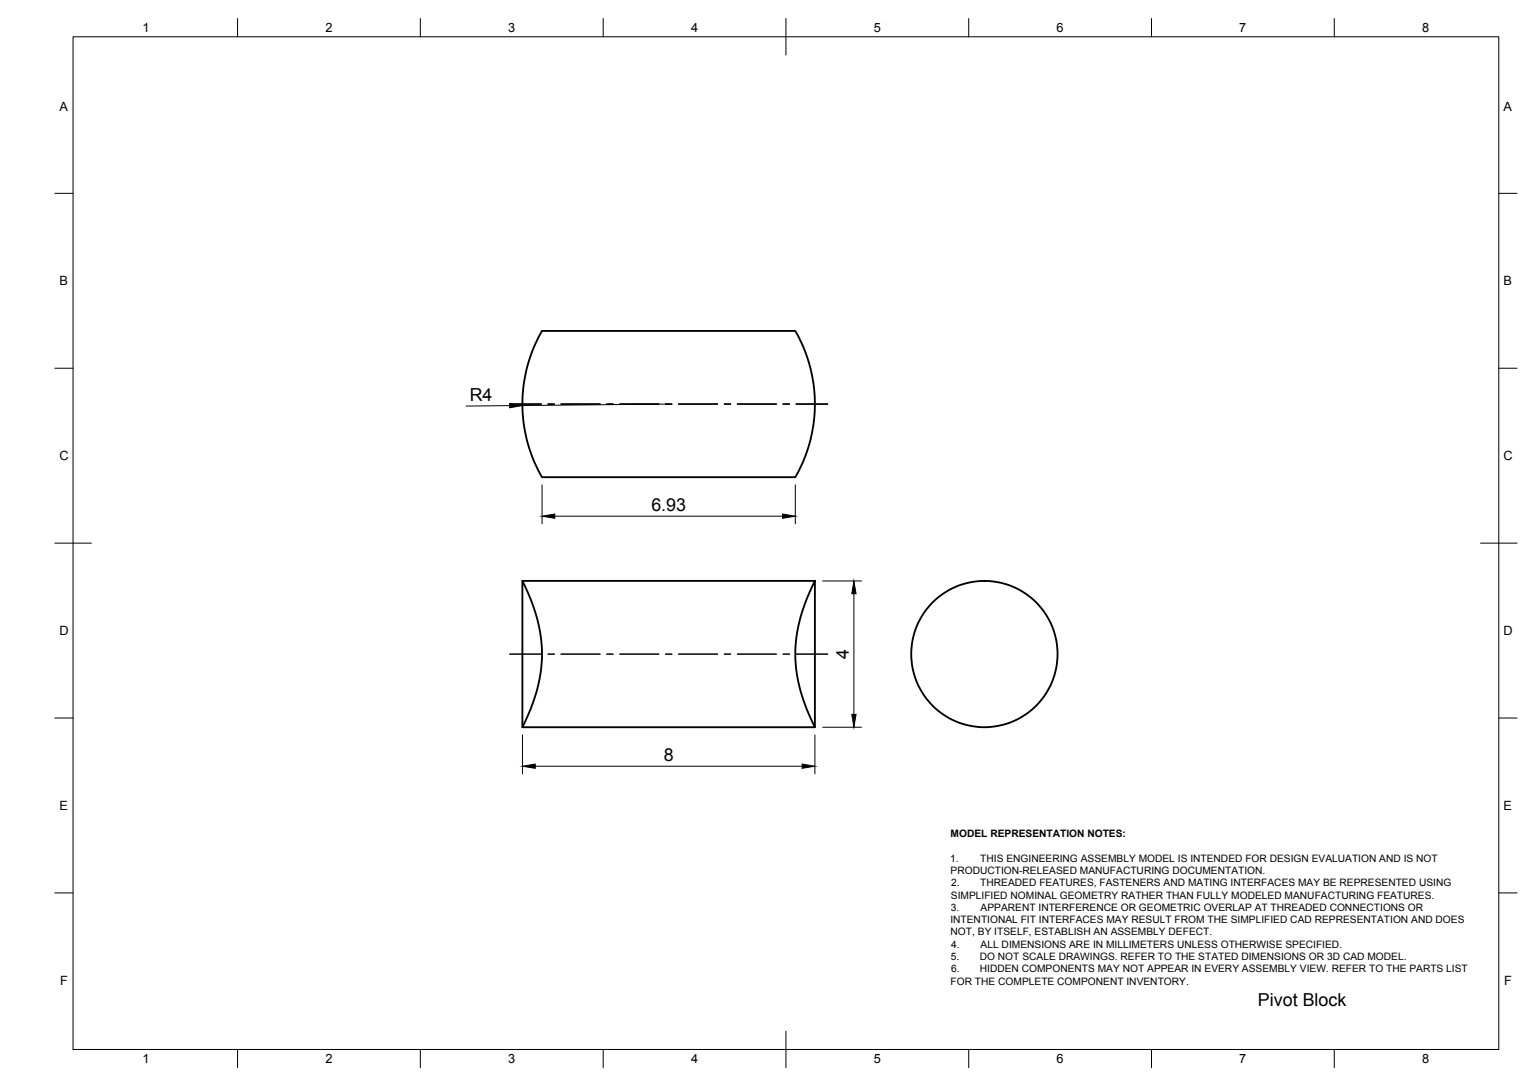
ISO-10303-21;
HEADER;
/* Generated by software containing ST-Developer
 * from STEP Tools, Inc. (www.steptools.com) 
 */

FILE_DESCRIPTION(
/* description */ ('STEP AP214'),
/* implementation_level */ '2;1');

FILE_NAME(
/* name */ 'Pivot Block.step',
/* time_stamp */ '2026-10-06T11:11:25-07:00',
/* author */ (''),
/* organization */ (''),
/* preprocessor_version */ 'ST-DEVELOPER v20.2',
/* originating_system */ 'Autodesk Translation Framework v15.15.0.0',
/* authorisation */ '');

FILE_SCHEMA (('AUTOMOTIVE_DESIGN { 1 0 10303 214 3 1 1 }'));
ENDSEC;

DATA;
#10=MECHANICAL_DESIGN_GEOMETRIC_PRESENTATION_REPRESENTATION('',(#703),#47717);
#450=B_SPLINE_CURVE_WITH_KNOTS('',3,(#44279,#44280,#44281,#44282,#44283,
#44284,#44285,#44286,#44287,#44288,#44289,#44290,#44291,#44292,#44293,#44294,
#44295,#44296,#44297,#44298,#44299,#44300,#44301,#44302,#44303,#44304,#44305),
 .UNSPECIFIED.,.F.,.F.,(4,2,2,2,3,2,2,2,2,2,2,2,4),(0.922537325049047,0.999310505714261,
1.07608368637947,1.15306672655577,1.23004976673206,1.30703280690836,1.38401584708465,
1.46078902774986,1.53756220841508,1.61433538908029,1.69110856974551,1.7680916099218,
1.84507465009809),.UNSPECIFIED.);
#451=B_SPLINE_CURVE_WITH_KNOTS('',3,(#44306,#44307,#44308,#44309,#44310,
#44311,#44312,#44313,#44314,#44315),.UNSPECIFIED.,.F.,.F.,(4,2,2,2,4),(1.84507465009809,
1.92205769027439,1.99904073045068,2.0758139111159,2.15258709178111),
 .UNSPECIFIED.);
#452=B_SPLINE_CURVE_WITH_KNOTS('',3,(#44318,#44319,#44320,#44321,#44322,
#44323,#44324,#44325,#44326,#44327,#44328,#44329,#44330,#44331,#44332,#44333,
#44334,#44335,#44336,#44337,#44338,#44339,#44340,#44341,#44342,#44343,#44344,
#44345,#44346,#44347,#44348,#44349,#44350,#44351),.UNSPECIFIED.,.T.,.F.,
(4,2,2,2,2,2,2,2,2,2,2,2,2,2,2,2,4),(-1.23004976673206,-1.15306672655577,
-1.07608368637947,-0.999310505714261,-0.922537325049047,-0.845764144383833,
-0.76899096371862,-0.692007923542325,-0.615024883366031,-0.538041843189737,
-0.461058803013443,-0.384285622348229,-0.307512441683016,-0.230739261017802,
-0.153966080352588,-0.0769830401762941,0.),.UNSPECIFIED.);
#679=SHAPE_REPRESENTATION_RELATIONSHIP('SRR','None',#47766,#691);
#691=ADVANCED_BREP_SHAPE_REPRESENTATION('',(#715),#47710);
#703=STYLED_ITEM('',(#47830),#715);
#715=MANIFOLD_SOLID_BREP('Body1',#8930);
#1145=LINE('',#44352,#1632);
#1632=VECTOR('',#11106,2.);
#1995=CYLINDRICAL_SURFACE('',#9512,4.);
#1996=CYLINDRICAL_SURFACE('',#9513,2.);
#1997=CYLINDRICAL_SURFACE('',#9514,4.);
#2360=FACE_OUTER_BOUND('',#2881,.T.);
#2361=FACE_OUTER_BOUND('',#2882,.T.);
#2362=FACE_OUTER_BOUND('',#2883,.T.);
#2881=EDGE_LOOP('',(#7339,#7340));
#2882=EDGE_LOOP('',(#7341,#7342,#7343,#7344,#7345));
#2883=EDGE_LOOP('',(#7346));
#4056=VERTEX_POINT('',#44277);
#4057=VERTEX_POINT('',#44278);
#4058=VERTEX_POINT('',#44317);
#5195=EDGE_CURVE('',#4056,#4057,#450,.T.);
#5196=EDGE_CURVE('',#4057,#4056,#451,.T.);
#5197=EDGE_CURVE('',#4058,#4058,#452,.T.);
#5198=EDGE_CURVE('',#4058,#4057,#1145,.T.);
#7339=ORIENTED_EDGE('',*,*,#5195,.T.);
#7340=ORIENTED_EDGE('',*,*,#5196,.T.);
#7341=ORIENTED_EDGE('',*,*,#5197,.F.);
#7342=ORIENTED_EDGE('',*,*,#5198,.T.);
#7343=ORIENTED_EDGE('',*,*,#5195,.F.);
#7344=ORIENTED_EDGE('',*,*,#5196,.F.);
#7345=ORIENTED_EDGE('',*,*,#5198,.F.);
#7346=ORIENTED_EDGE('',*,*,#5197,.T.);
#8710=ADVANCED_FACE('',(#2360),#1995,.T.);
#8711=ADVANCED_FACE('',(#2361),#1996,.T.);
#8712=ADVANCED_FACE('',(#2362),#1997,.T.);
#8930=CLOSED_SHELL('',(#8710,#8711,#8712));
#9511=AXIS2_PLACEMENT_3D('',#44275,#11100,#11101);
#9512=AXIS2_PLACEMENT_3D('',#44276,#11102,#11103);
#9513=AXIS2_PLACEMENT_3D('',#44316,#11104,#11105);
#9514=AXIS2_PLACEMENT_3D('',#44353,#11107,#11108);
#11100=DIRECTION('axis',(0.,0.,1.));
#11101=DIRECTION('refdir',(1.,0.,0.));
#11102=DIRECTION('center_axis',(0.106006004448152,0.994365489657067,0.));
#11103=DIRECTION('ref_axis',(0.,0.,1.));
#11104=DIRECTION('center_axis',(0.,0.,-1.));
#11105=DIRECTION('ref_axis',(-0.994365489657067,0.106006004448153,0.));
#11106=DIRECTION('',(0.,0.,1.));
#11107=DIRECTION('center_axis',(0.106006004448152,0.994365489657067,0.));
#11108=DIRECTION('ref_axis',(1.21774651409112E-16,-1.29819914037829E-17,
-1.));
#44275=CARTESIAN_POINT('',(0.,0.,0.));
#44276=CARTESIAN_POINT('Origin',(-53.8258982150057,-64.4396735761727,175.985485069079));
#44277=CARTESIAN_POINT('',(-53.4018741972131,-60.4622116175444,179.985485069079));
#44278=CARTESIAN_POINT('',(-51.6251552267953,-62.6629546057548,179.449586684217));
#44279=CARTESIAN_POINT('Ctrl Pts',(-53.4018741972131,-60.4622116175444,
179.985485069079));
#44280=CARTESIAN_POINT('Ctrl Pts',(-53.6563428684955,-60.4350835571074,
179.985485069079));
#44281=CARTESIAN_POINT('Ctrl Pts',(-53.9303211793164,-60.458242890839,179.958669005781));
#44282=CARTESIAN_POINT('Ctrl Pts',(-54.4409372535361,-60.6105704641806,
179.862014751158));
#44283=CARTESIAN_POINT('Ctrl Pts',(-54.6778490486358,-60.7394791031505,
179.79321828922));
#44284=CARTESIAN_POINT('Ctrl Pts',(-55.0631092638411,-61.0505100306915,
179.660886004177));
#44285=CARTESIAN_POINT('Ctrl Pts',(-55.2387001635013,-61.2547981540133,
179.587877094001));
#44286=CARTESIAN_POINT('Ctrl Pts',(-55.4948940947938,-61.7211552694728,
179.481135940985));
#44287=CARTESIAN_POINT('Ctrl Pts',(-55.5754149704257,-61.9837663264949,
179.449586684217));
#44288=CARTESIAN_POINT('Ctrl Pts',(-55.6026171854236,-62.2389305879622,
179.449586684217));
#44289=CARTESIAN_POINT('Ctrl Pts',(-55.6298194004214,-62.4940948494295,
179.449586684217));
#44290=CARTESIAN_POINT('Ctrl Pts',(-55.6064711817378,-62.7677790458441,
179.481135940985));
#44291=CARTESIAN_POINT('Ctrl Pts',(-55.4543512989582,-63.2776651417851,
179.587877094001));
#44292=CARTESIAN_POINT('Ctrl Pts',(-55.3257742211671,-63.5143796036173,
179.660886004177));
#44293=CARTESIAN_POINT('Ctrl Pts',(-55.0147432936261,-63.8996398188226,
179.79321828922));
#44294=CARTESIAN_POINT('Ctrl Pts',(-54.8103321708864,-64.0755964292659,
179.862014751158));
#44295=CARTESIAN_POINT('Ctrl Pts',(-54.343305267868,-64.3321472755105,179.958669005781));
#44296=CARTESIAN_POINT('Ctrl Pts',(-54.080366886288,-64.4125455157357,179.985485069079));
#44297=CARTESIAN_POINT('Ctrl Pts',(-53.5714295437234,-64.4668016366096,
179.985485069079));
#44298=CARTESIAN_POINT('Ctrl Pts',(-53.2974512329025,-64.443642302878,179.958669005781));
#44299=CARTESIAN_POINT('Ctrl Pts',(-52.7868351586827,-64.2913147295365,
179.862014751158));
#44300=CARTESIAN_POINT('Ctrl Pts',(-52.549923363583,-64.1624060905666,179.79321828922));
#44301=CARTESIAN_POINT('Ctrl Pts',(-52.1646631483778,-63.8513751630256,
179.660886004177));
#44302=CARTESIAN_POINT('Ctrl Pts',(-51.9890722487176,-63.6470870397037,
179.587877094001));
#44303=CARTESIAN_POINT('Ctrl Pts',(-51.732878317425,-63.1807299242443,179.481135940985));
#44304=CARTESIAN_POINT('Ctrl Pts',(-51.6523574417932,-62.9181188672221,
179.449586684217));
#44305=CARTESIAN_POINT('Ctrl Pts',(-51.6251552267953,-62.6629546057548,
179.449586684217));
#44306=CARTESIAN_POINT('Ctrl Pts',(-51.6251552267953,-62.6629546057548,
179.449586684217));
#44307=CARTESIAN_POINT('Ctrl Pts',(-51.5979530117974,-62.4077903442875,
179.449586684217));
#44308=CARTESIAN_POINT('Ctrl Pts',(-51.6213012304811,-62.1341061478729,
179.481135940985));
#44309=CARTESIAN_POINT('Ctrl Pts',(-51.7734211132606,-61.6242200519319,
179.587877094001));
#44310=CARTESIAN_POINT('Ctrl Pts',(-51.9019981910518,-61.3875055900997,
179.660886004177));
#44311=CARTESIAN_POINT('Ctrl Pts',(-52.2130291185928,-61.0022453748944,
179.79321828922));
#44312=CARTESIAN_POINT('Ctrl Pts',(-52.4174402413325,-60.8262887644511,
179.862014751158));
#44313=CARTESIAN_POINT('Ctrl Pts',(-52.8844671443509,-60.5697379182066,
179.958669005781));
#44314=CARTESIAN_POINT('Ctrl Pts',(-53.1474055259308,-60.4893396779814,
179.985485069079));
#44315=CARTESIAN_POINT('Ctrl Pts',(-53.4018741972131,-60.4622116175444,
179.985485069079));
#44316=CARTESIAN_POINT('Origin',(-53.6138862061094,-62.4509425968585,185.985485069079));
#44317=CARTESIAN_POINT('',(-51.6251552267953,-62.6629546057548,172.521383453942));
#44318=CARTESIAN_POINT('Ctrl Pts',(-55.6026171854236,-62.2389305879622,
172.521383453942));
#44319=CARTESIAN_POINT('Ctrl Pts',(-55.5754149704257,-61.9837663264949,
172.521383453942));
#44320=CARTESIAN_POINT('Ctrl Pts',(-55.4948940947938,-61.7211552694728,
172.489834197174));
#44321=CARTESIAN_POINT('Ctrl Pts',(-55.2387001635013,-61.2547981540133,
172.383093044158));
#44322=CARTESIAN_POINT('Ctrl Pts',(-55.0631092638411,-61.0505100306915,
172.310084133982));
#44323=CARTESIAN_POINT('Ctrl Pts',(-54.6778490486358,-60.7394791031505,
172.177751848938));
#44324=CARTESIAN_POINT('Ctrl Pts',(-54.4409372535361,-60.6105704641806,
172.108955387));
#44325=CARTESIAN_POINT('Ctrl Pts',(-53.9303211793164,-60.458242890839,172.012301132378));
#44326=CARTESIAN_POINT('Ctrl Pts',(-53.6563428684955,-60.4350835571074,
171.985485069079));
#44327=CARTESIAN_POINT('Ctrl Pts',(-53.1474055259308,-60.4893396779814,
171.985485069079));
#44328=CARTESIAN_POINT('Ctrl Pts',(-52.8844671443509,-60.5697379182066,
172.012301132378));
#44329=CARTESIAN_POINT('Ctrl Pts',(-52.4174402413325,-60.8262887644511,
172.108955387));
#44330=CARTESIAN_POINT('Ctrl Pts',(-52.2130291185928,-61.0022453748944,
172.177751848938));
#44331=CARTESIAN_POINT('Ctrl Pts',(-51.9019981910518,-61.3875055900997,
172.310084133982));
#44332=CARTESIAN_POINT('Ctrl Pts',(-51.7734211132606,-61.6242200519319,
172.383093044158));
#44333=CARTESIAN_POINT('Ctrl Pts',(-51.6213012304811,-62.1341061478729,
172.489834197174));
#44334=CARTESIAN_POINT('Ctrl Pts',(-51.5979530117974,-62.4077903442875,
172.521383453942));
#44335=CARTESIAN_POINT('Ctrl Pts',(-51.6523574417932,-62.9181188672221,
172.521383453942));
#44336=CARTESIAN_POINT('Ctrl Pts',(-51.732878317425,-63.1807299242443,172.489834197174));
#44337=CARTESIAN_POINT('Ctrl Pts',(-51.9890722487176,-63.6470870397037,
172.383093044158));
#44338=CARTESIAN_POINT('Ctrl Pts',(-52.1646631483778,-63.8513751630256,
172.310084133982));
#44339=CARTESIAN_POINT('Ctrl Pts',(-52.549923363583,-64.1624060905665,172.177751848938));
#44340=CARTESIAN_POINT('Ctrl Pts',(-52.7868351586827,-64.2913147295365,
172.108955387));
#44341=CARTESIAN_POINT('Ctrl Pts',(-53.2974512329024,-64.443642302878,172.012301132378));
#44342=CARTESIAN_POINT('Ctrl Pts',(-53.5714295437234,-64.4668016366096,
171.985485069079));
#44343=CARTESIAN_POINT('Ctrl Pts',(-54.080366886288,-64.4125455157357,171.985485069079));
#44344=CARTESIAN_POINT('Ctrl Pts',(-54.343305267868,-64.3321472755105,172.012301132378));
#44345=CARTESIAN_POINT('Ctrl Pts',(-54.8103321708864,-64.0755964292659,
172.108955387));
#44346=CARTESIAN_POINT('Ctrl Pts',(-55.0147432936261,-63.8996398188226,
172.177751848938));
#44347=CARTESIAN_POINT('Ctrl Pts',(-55.3257742211671,-63.5143796036173,
172.310084133982));
#44348=CARTESIAN_POINT('Ctrl Pts',(-55.4543512989582,-63.2776651417851,
172.383093044158));
#44349=CARTESIAN_POINT('Ctrl Pts',(-55.6064711817378,-62.7677790458441,
172.489834197174));
#44350=CARTESIAN_POINT('Ctrl Pts',(-55.6298194004214,-62.4940948494295,
172.521383453942));
#44351=CARTESIAN_POINT('Ctrl Pts',(-55.6026171854236,-62.2389305879622,
172.521383453942));
#44352=CARTESIAN_POINT('',(-51.6251552267953,-62.6629546057548,185.985485069079));
#44353=CARTESIAN_POINT('Origin',(-53.8258982150057,-64.4396735761727,175.985485069079));
#47696=UNCERTAINTY_MEASURE_WITH_UNIT(LENGTH_MEASURE(0.01),#47718,
'DISTANCE_ACCURACY_VALUE',
'Maximum model space distance between geometric entities at asserted c
onnectivities');
#47703=UNCERTAINTY_MEASURE_WITH_UNIT(LENGTH_MEASURE(0.01),#47718,
'DISTANCE_ACCURACY_VALUE',
'Maximum model space distance between geometric entities at asserted c
onnectivities');
#47710=(
GEOMETRIC_REPRESENTATION_CONTEXT(3)
GLOBAL_UNCERTAINTY_ASSIGNED_CONTEXT((#47696))
GLOBAL_UNIT_ASSIGNED_CONTEXT((#47718,#47720,#47721))
REPRESENTATION_CONTEXT('','3D')
);
#47717=(
GEOMETRIC_REPRESENTATION_CONTEXT(3)
GLOBAL_UNCERTAINTY_ASSIGNED_CONTEXT((#47703))
GLOBAL_UNIT_ASSIGNED_CONTEXT((#47718,#47720,#47721))
REPRESENTATION_CONTEXT('','3D')
);
#47718=(
LENGTH_UNIT()
NAMED_UNIT(*)
SI_UNIT(.MILLI.,.METRE.)
);
#47720=(
NAMED_UNIT(*)
PLANE_ANGLE_UNIT()
SI_UNIT($,.RADIAN.)
);
#47721=(
NAMED_UNIT(*)
SI_UNIT($,.STERADIAN.)
SOLID_ANGLE_UNIT()
);
#47728=SHAPE_DEFINITION_REPRESENTATION(#47741,#47766);
#47741=PRODUCT_DEFINITION_SHAPE('',$,#47780);
#47766=SHAPE_REPRESENTATION('',(#9511),#47710);
#47773=PRODUCT_DEFINITION_CONTEXT('part definition',#47814,'design');
#47780=PRODUCT_DEFINITION('Pivot Block','Pivot Block',#47793,#47773);
#47793=PRODUCT_DEFINITION_FORMATION('',$,#47822);
#47814=APPLICATION_CONTEXT(
'Core Data for Automotive Mechanical Design Process');
#47815=PRODUCT_CONTEXT('part definition',#47814,'mechanical');
#47822=PRODUCT('Pivot Block','Pivot Block',$,(#47815));
#47830=PRESENTATION_STYLE_ASSIGNMENT((#47832));
#47832=SURFACE_STYLE_USAGE(.BOTH.,#47834);
#47834=SURFACE_SIDE_STYLE('',(#47836));
#47836=SURFACE_STYLE_FILL_AREA(#47838);
#47838=FILL_AREA_STYLE('Opaque(202,209,238)',(#47840));
#47840=FILL_AREA_STYLE_COLOUR('Opaque(202,209,238)',#47842);
#47842=COLOUR_RGB('Opaque(202,209,238)', 0.66274510, 0.83137255, 0.94901961);
ENDSEC;
END-ISO-10303-21;
